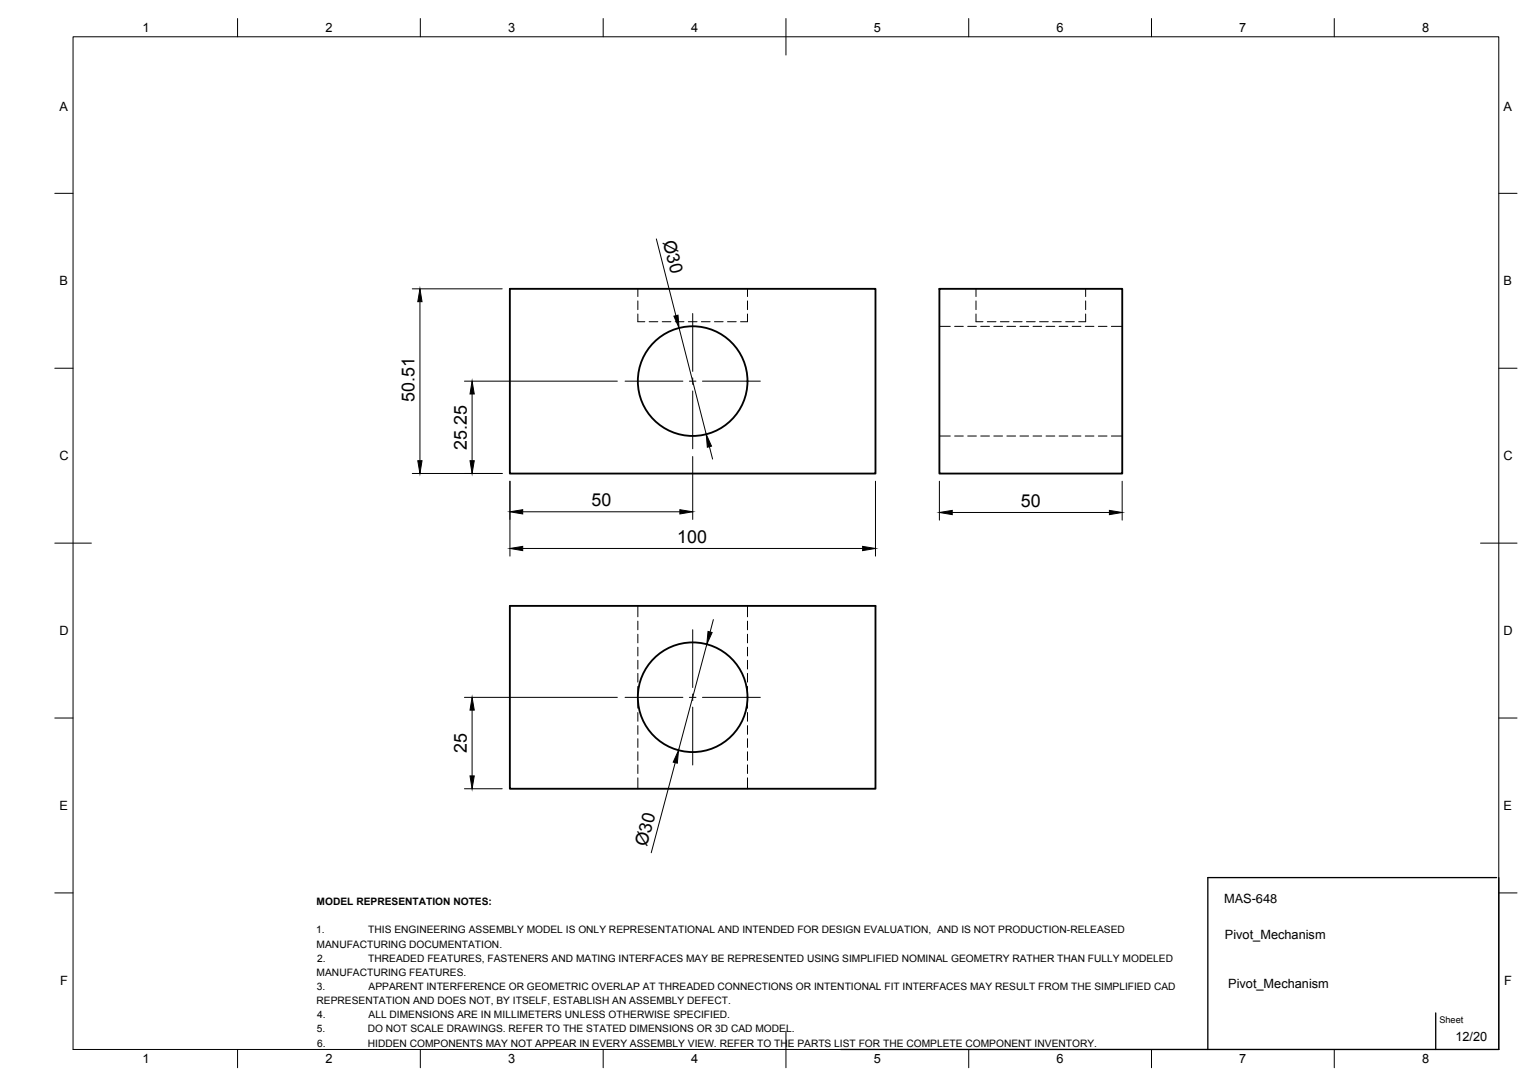
ISO-10303-21;
HEADER;
FILE_DESCRIPTION((''),'2;1');
FILE_NAME('Pivot_Mechanism.step','2026-10-09T12:47:58-07:00',(''),(''),'','','');
FILE_SCHEMA (('AUTOMOTIVE_DESIGN { 1 0 10303 214 3 1 1 }'));
ENDSEC;
DATA;
#10=MECHANICAL_DESIGN_GEOMETRIC_PRESENTATION_REPRESENTATION('',(#315),#3475);
#148=FACE_BOUND('',#494,.T.) ;
#149=FACE_BOUND('',#497,.T.) ;
#150=FACE_BOUND('',#499,.T.) ;
#178=CIRCLE('',#2031,15.) ;
#179=CIRCLE('',#2032,15.) ;
#180=CIRCLE('',#2034,15.) ;
#181=CIRCLE('',#2035,15.) ;
#263=CYLINDRICAL_SURFACE('',#2030,15.) ;
#264=CYLINDRICAL_SURFACE('',#2033,15.) ;
#291=SHAPE_REPRESENTATION_RELATIONSHIP('SRR','None',#3546,#303) ;
#303=ADVANCED_BREP_SHAPE_REPRESENTATION('',(#327),#3466) ;
#315=STYLED_ITEM('',(#3628),#327) ;
#327=MANIFOLD_SOLID_BREP('Body1',#1829) ;
#370=FACE_OUTER_BOUND('',#491,.T.) ;
#371=FACE_OUTER_BOUND('',#492,.T.) ;
#372=FACE_OUTER_BOUND('',#493,.T.) ;
#373=FACE_OUTER_BOUND('',#495,.T.) ;
#374=FACE_OUTER_BOUND('',#496,.T.) ;
#375=FACE_OUTER_BOUND('',#498,.T.) ;
#376=FACE_OUTER_BOUND('',#500,.T.) ;
#377=FACE_OUTER_BOUND('',#501,.T.) ;
#378=FACE_OUTER_BOUND('',#502,.T.) ;
#491=EDGE_LOOP('',(#1352,#1353,#1354,#1355)) ;
#492=EDGE_LOOP('',(#1356,#1357,#1358,#1359)) ;
#493=EDGE_LOOP('',(#1360,#1361,#1362,#1363)) ;
#494=EDGE_LOOP('',(#1364)) ;
#495=EDGE_LOOP('',(#1365,#1366,#1367,#1368)) ;
#496=EDGE_LOOP('',(#1369,#1370,#1371,#1372)) ;
#497=EDGE_LOOP('',(#1373)) ;
#498=EDGE_LOOP('',(#1374,#1375,#1376,#1377)) ;
#499=EDGE_LOOP('',(#1378)) ;
#500=EDGE_LOOP('',(#1379,#1380,#1381,#1382)) ;
#501=EDGE_LOOP('',(#1383,#1384,#1385,#1386)) ;
#502=EDGE_LOOP('',(#1387)) ;
#650=LINE('',#3076,#769) ;
#651=LINE('',#3082,#770) ;
#652=LINE('',#3087,#771) ;
#653=LINE('',#3089,#772) ;
#654=LINE('',#3091,#773) ;
#655=LINE('',#3092,#774) ;
#656=LINE('',#3095,#775) ;
#657=LINE('',#3097,#776) ;
#658=LINE('',#3098,#777) ;
#659=LINE('',#3101,#778) ;
#660=LINE('',#3103,#779) ;
#661=LINE('',#3104,#780) ;
#662=LINE('',#3106,#781) ;
#663=LINE('',#3107,#782) ;
#769=VECTOR('',#2403,15.) ;
#770=VECTOR('',#2410,15.) ;
#771=VECTOR('',#2415,1000.) ;
#772=VECTOR('',#2416,1000.) ;
#773=VECTOR('',#2417,1000.) ;
#774=VECTOR('',#2418,1000.) ;
#775=VECTOR('',#2421,1000.) ;
#776=VECTOR('',#2422,1000.) ;
#777=VECTOR('',#2423,1000.) ;
#778=VECTOR('',#2426,1000.) ;
#779=VECTOR('',#2427,1000.) ;
#780=VECTOR('',#2428,1000.) ;
#781=VECTOR('',#2431,1000.) ;
#782=VECTOR('',#2432,1000.) ;
#877=VERTEX_POINT('',#3073) ;
#878=VERTEX_POINT('',#3075) ;
#879=VERTEX_POINT('',#3079) ;
#880=VERTEX_POINT('',#3081) ;
#881=VERTEX_POINT('',#3085) ;
#882=VERTEX_POINT('',#3086) ;
#883=VERTEX_POINT('',#3088) ;
#884=VERTEX_POINT('',#3090) ;
#885=VERTEX_POINT('',#3094) ;
#886=VERTEX_POINT('',#3096) ;
#887=VERTEX_POINT('',#3100) ;
#888=VERTEX_POINT('',#3102) ;
#1048=EDGE_CURVE('',#877,#877,#178,.T.) ;
#1049=EDGE_CURVE('',#877,#878,#650,.T.) ;
#1050=EDGE_CURVE('',#878,#878,#179,.T.) ;
#1051=EDGE_CURVE('',#879,#879,#180,.T.) ;
#1052=EDGE_CURVE('',#879,#880,#651,.T.) ;
#1053=EDGE_CURVE('',#880,#880,#181,.T.) ;
#1054=EDGE_CURVE('',#881,#882,#652,.T.) ;
#1055=EDGE_CURVE('',#883,#882,#653,.T.) ;
#1056=EDGE_CURVE('',#884,#883,#654,.T.) ;
#1057=EDGE_CURVE('',#884,#881,#655,.T.) ;
#1058=EDGE_CURVE('',#882,#885,#656,.T.) ;
#1059=EDGE_CURVE('',#886,#885,#657,.T.) ;
#1060=EDGE_CURVE('',#883,#886,#658,.T.) ;
#1061=EDGE_CURVE('',#885,#887,#659,.T.) ;
#1062=EDGE_CURVE('',#888,#887,#660,.T.) ;
#1063=EDGE_CURVE('',#886,#888,#661,.T.) ;
#1064=EDGE_CURVE('',#887,#881,#662,.T.) ;
#1065=EDGE_CURVE('',#888,#884,#663,.T.) ;
#1352=ORIENTED_EDGE('',*,*,#1048,.F.) ;
#1353=ORIENTED_EDGE('',*,*,#1049,.T.) ;
#1354=ORIENTED_EDGE('',*,*,#1050,.T.) ;
#1355=ORIENTED_EDGE('',*,*,#1049,.F.) ;
#1356=ORIENTED_EDGE('',*,*,#1051,.F.) ;
#1357=ORIENTED_EDGE('',*,*,#1052,.T.) ;
#1358=ORIENTED_EDGE('',*,*,#1053,.T.) ;
#1359=ORIENTED_EDGE('',*,*,#1052,.F.) ;
#1360=ORIENTED_EDGE('',*,*,#1054,.T.) ;
#1361=ORIENTED_EDGE('',*,*,#1055,.F.) ;
#1362=ORIENTED_EDGE('',*,*,#1056,.F.) ;
#1363=ORIENTED_EDGE('',*,*,#1057,.T.) ;
#1364=ORIENTED_EDGE('',*,*,#1048,.T.) ;
#1365=ORIENTED_EDGE('',*,*,#1058,.T.) ;
#1366=ORIENTED_EDGE('',*,*,#1059,.F.) ;
#1367=ORIENTED_EDGE('',*,*,#1060,.F.) ;
#1368=ORIENTED_EDGE('',*,*,#1055,.T.) ;
#1369=ORIENTED_EDGE('',*,*,#1061,.T.) ;
#1370=ORIENTED_EDGE('',*,*,#1062,.F.) ;
#1371=ORIENTED_EDGE('',*,*,#1063,.F.) ;
#1372=ORIENTED_EDGE('',*,*,#1059,.T.) ;
#1373=ORIENTED_EDGE('',*,*,#1050,.F.) ;
#1374=ORIENTED_EDGE('',*,*,#1064,.T.) ;
#1375=ORIENTED_EDGE('',*,*,#1057,.F.) ;
#1376=ORIENTED_EDGE('',*,*,#1065,.F.) ;
#1377=ORIENTED_EDGE('',*,*,#1062,.T.) ;
#1378=ORIENTED_EDGE('',*,*,#1053,.F.) ;
#1379=ORIENTED_EDGE('',*,*,#1056,.T.) ;
#1380=ORIENTED_EDGE('',*,*,#1060,.T.) ;
#1381=ORIENTED_EDGE('',*,*,#1063,.T.) ;
#1382=ORIENTED_EDGE('',*,*,#1065,.T.) ;
#1383=ORIENTED_EDGE('',*,*,#1054,.F.) ;
#1384=ORIENTED_EDGE('',*,*,#1064,.F.) ;
#1385=ORIENTED_EDGE('',*,*,#1061,.F.) ;
#1386=ORIENTED_EDGE('',*,*,#1058,.F.) ;
#1387=ORIENTED_EDGE('',*,*,#1051,.T.) ;
#1672=PLANE('',#2036) ;
#1673=PLANE('',#2037) ;
#1674=PLANE('',#2038) ;
#1675=PLANE('',#2039) ;
#1676=PLANE('',#2040) ;
#1677=PLANE('',#2041) ;
#1678=PLANE('',#2042) ;
#1746=ADVANCED_FACE('',(#370),#263,.F.) ;
#1747=ADVANCED_FACE('',(#371),#264,.F.) ;
#1748=ADVANCED_FACE('',(#372,#148),#1672,.F.) ;
#1749=ADVANCED_FACE('',(#373),#1673,.F.) ;
#1750=ADVANCED_FACE('',(#374,#149),#1674,.F.) ;
#1751=ADVANCED_FACE('',(#375,#150),#1675,.F.) ;
#1752=ADVANCED_FACE('',(#376),#1676,.T.) ;
#1753=ADVANCED_FACE('',(#377),#1677,.F.) ;
#1754=ADVANCED_FACE('',(#378),#1678,.T.) ;
#1829=CLOSED_SHELL('',(#1746,#1747,#1748,#1749,#1750,#1751,#1752,#1753,
#1754)) ;
#2029=AXIS2_PLACEMENT_3D('',#3071,#2397,#2398) ;
#2030=AXIS2_PLACEMENT_3D('',#3072,#2399,#2400) ;
#2031=AXIS2_PLACEMENT_3D('',#3074,#2401,#2402) ;
#2032=AXIS2_PLACEMENT_3D('',#3077,#2404,#2405) ;
#2033=AXIS2_PLACEMENT_3D('',#3078,#2406,#2407) ;
#2034=AXIS2_PLACEMENT_3D('',#3080,#2408,#2409) ;
#2035=AXIS2_PLACEMENT_3D('',#3083,#2411,#2412) ;
#2036=AXIS2_PLACEMENT_3D('',#3084,#2413,#2414) ;
#2037=AXIS2_PLACEMENT_3D('',#3093,#2419,#2420) ;
#2038=AXIS2_PLACEMENT_3D('',#3099,#2424,#2425) ;
#2039=AXIS2_PLACEMENT_3D('',#3105,#2429,#2430) ;
#2040=AXIS2_PLACEMENT_3D('',#3108,#2433,#2434) ;
#2041=AXIS2_PLACEMENT_3D('',#3109,#2435,#2436) ;
#2042=AXIS2_PLACEMENT_3D('',#3110,#2437,#2438) ;
#2397=DIRECTION('axis',(0.,0.,1.)) ;
#2398=DIRECTION('refdir',(1.,0.,0.)) ;
#2399=DIRECTION('center_axis',(1.,0.,0.)) ;
#2400=DIRECTION('ref_axis',(0.,0.,-1.)) ;
#2401=DIRECTION('center_axis',(1.,0.,0.)) ;
#2402=DIRECTION('ref_axis',(0.,0.,-1.)) ;
#2403=DIRECTION('',(1.,0.,0.)) ;
#2404=DIRECTION('center_axis',(1.,0.,0.)) ;
#2405=DIRECTION('ref_axis',(0.,0.,-1.)) ;
#2406=DIRECTION('center_axis',(0.,1.,0.)) ;
#2407=DIRECTION('ref_axis',(0.,0.,1.)) ;
#2408=DIRECTION('center_axis',(0.,1.,0.)) ;
#2409=DIRECTION('ref_axis',(0.,0.,1.)) ;
#2410=DIRECTION('',(0.,1.,0.)) ;
#2411=DIRECTION('center_axis',(0.,1.,0.)) ;
#2412=DIRECTION('ref_axis',(0.,0.,1.)) ;
#2413=DIRECTION('center_axis',(1.,0.,0.)) ;
#2414=DIRECTION('ref_axis',(0.,0.,-1.)) ;
#2415=DIRECTION('',(0.,-1.,0.)) ;
#2416=DIRECTION('',(0.,0.,-1.)) ;
#2417=DIRECTION('',(0.,-1.,0.)) ;
#2418=DIRECTION('',(0.,0.,-1.)) ;
#2419=DIRECTION('center_axis',(0.,1.,0.)) ;
#2420=DIRECTION('ref_axis',(0.,0.,1.)) ;
#2421=DIRECTION('',(1.,0.,0.)) ;
#2422=DIRECTION('',(0.,0.,-1.)) ;
#2423=DIRECTION('',(1.,0.,0.)) ;
#2424=DIRECTION('center_axis',(-1.,0.,0.)) ;
#2425=DIRECTION('ref_axis',(0.,0.,1.)) ;
#2426=DIRECTION('',(0.,1.,0.)) ;
#2427=DIRECTION('',(0.,0.,-1.)) ;
#2428=DIRECTION('',(0.,1.,0.)) ;
#2429=DIRECTION('center_axis',(0.,-1.,0.)) ;
#2430=DIRECTION('ref_axis',(0.,0.,-1.)) ;
#2431=DIRECTION('',(-1.,0.,0.)) ;
#2432=DIRECTION('',(-1.,0.,0.)) ;
#2433=DIRECTION('center_axis',(0.,0.,1.)) ;
#2434=DIRECTION('ref_axis',(1.,0.,0.)) ;
#2435=DIRECTION('center_axis',(0.,0.,1.)) ;
#2436=DIRECTION('ref_axis',(1.,0.,0.)) ;
#2437=DIRECTION('center_axis',(0.,1.,0.)) ;
#2438=DIRECTION('ref_axis',(0.,0.,1.)) ;
#3071=CARTESIAN_POINT('',(0.,0.,0.)) ;
#3072=CARTESIAN_POINT('Origin',(-25.,0.,0.)) ;
#3073=CARTESIAN_POINT('',(-25.,-1.83697019872103E-15,15.)) ;
#3074=CARTESIAN_POINT('Origin',(-25.,0.,0.)) ;
#3075=CARTESIAN_POINT('',(25.,-1.83697019872103E-15,15.)) ;
#3076=CARTESIAN_POINT('',(-25.,-1.83697019872103E-15,15.)) ;
#3077=CARTESIAN_POINT('Origin',(25.,0.,0.)) ;
#3078=CARTESIAN_POINT('Origin',(0.,16.254058593968,0.)) ;
#3079=CARTESIAN_POINT('',(-1.83697019872103E-15,16.254058593968,-15.)) ;
#3080=CARTESIAN_POINT('Origin',(0.,16.254058593968,0.)) ;
#3081=CARTESIAN_POINT('',(-1.83697019872103E-15,25.254058593968,-15.)) ;
#3082=CARTESIAN_POINT('',(-1.83697019872103E-15,16.254058593968,-15.)) ;
#3083=CARTESIAN_POINT('Origin',(0.,25.254058593968,0.)) ;
#3084=CARTESIAN_POINT('Origin',(-25.,-25.254058593968,50.)) ;
#3085=CARTESIAN_POINT('',(-25.,25.254058593968,-50.)) ;
#3086=CARTESIAN_POINT('',(-25.,-25.254058593968,-50.)) ;
#3087=CARTESIAN_POINT('',(-25.,-25.254058593968,-50.)) ;
#3088=CARTESIAN_POINT('',(-25.,-25.254058593968,50.)) ;
#3089=CARTESIAN_POINT('',(-25.,-25.254058593968,50.)) ;
#3090=CARTESIAN_POINT('',(-25.,25.254058593968,50.)) ;
#3091=CARTESIAN_POINT('',(-25.,-25.254058593968,50.)) ;
#3092=CARTESIAN_POINT('',(-25.,25.254058593968,50.)) ;
#3093=CARTESIAN_POINT('Origin',(25.,-25.254058593968,50.)) ;
#3094=CARTESIAN_POINT('',(25.,-25.254058593968,-50.)) ;
#3095=CARTESIAN_POINT('',(25.,-25.254058593968,-50.)) ;
#3096=CARTESIAN_POINT('',(25.,-25.254058593968,50.)) ;
#3097=CARTESIAN_POINT('',(25.,-25.254058593968,50.)) ;
#3098=CARTESIAN_POINT('',(25.,-25.254058593968,50.)) ;
#3099=CARTESIAN_POINT('Origin',(25.,-25.254058593968,50.)) ;
#3100=CARTESIAN_POINT('',(25.,25.254058593968,-50.)) ;
#3101=CARTESIAN_POINT('',(25.,-25.254058593968,-50.)) ;
#3102=CARTESIAN_POINT('',(25.,25.254058593968,50.)) ;
#3103=CARTESIAN_POINT('',(25.,25.254058593968,50.)) ;
#3104=CARTESIAN_POINT('',(25.,-25.254058593968,50.)) ;
#3105=CARTESIAN_POINT('Origin',(25.,25.254058593968,50.)) ;
#3106=CARTESIAN_POINT('',(25.,25.254058593968,-50.)) ;
#3107=CARTESIAN_POINT('',(25.,25.254058593968,50.)) ;
#3108=CARTESIAN_POINT('Origin',(0.,0.,50.)) ;
#3109=CARTESIAN_POINT('Origin',(0.,0.,-50.)) ;
#3110=CARTESIAN_POINT('Origin',(0.,16.254058593968,0.)) ;
#3448=UNCERTAINTY_MEASURE_WITH_UNIT(LENGTH_MEASURE(0.01),#3476,
'DISTANCE_ACCURACY_VALUE',
'Maximum model space distance between geometric entities at asserted c
onnectivities') ;
#3457=UNCERTAINTY_MEASURE_WITH_UNIT(LENGTH_MEASURE(0.01),#3476,
'DISTANCE_ACCURACY_VALUE',
'Maximum model space distance between geometric entities at asserted c
onnectivities') ;
#3466=(
GEOMETRIC_REPRESENTATION_CONTEXT(3)
GLOBAL_UNCERTAINTY_ASSIGNED_CONTEXT((#3448))
GLOBAL_UNIT_ASSIGNED_CONTEXT((#3476,#3478,#3479))
REPRESENTATION_CONTEXT('','3D')
) ;
#3475=(
GEOMETRIC_REPRESENTATION_CONTEXT(3)
GLOBAL_UNCERTAINTY_ASSIGNED_CONTEXT((#3457))
GLOBAL_UNIT_ASSIGNED_CONTEXT((#3476,#3478,#3479))
REPRESENTATION_CONTEXT('','3D')
) ;
#3476=(
LENGTH_UNIT()
NAMED_UNIT(*)
SI_UNIT(.MILLI.,.METRE.)
) ;
#3478=(
NAMED_UNIT(*)
PLANE_ANGLE_UNIT()
SI_UNIT($,.RADIAN.)
) ;
#3479=(
NAMED_UNIT(*)
SI_UNIT($,.STERADIAN.)
SOLID_ANGLE_UNIT()
) ;
#3488=SHAPE_DEFINITION_REPRESENTATION(#3509,#3546) ;
#3509=PRODUCT_DEFINITION_SHAPE('',$,#3564) ;
#3546=SHAPE_REPRESENTATION('',(#2029),#3466) ;
#3555=PRODUCT_DEFINITION_CONTEXT('part definition',#3608,'design') ;
#3564=PRODUCT_DEFINITION('Pivot_Mechanism','Pivot_Mechanism',#3581,#3555) ;
#3581=PRODUCT_DEFINITION_FORMATION('',$,#3618) ;
#3608=APPLICATION_CONTEXT(
'Core Data for Automotive Mechanical Design Process') ;
#3609=PRODUCT_CONTEXT('part definition',#3608,'mechanical') ;
#3618=PRODUCT('Pivot_Mechanism',
'Pivot_Mechanism',$,(#3609)) ;
#3628=PRESENTATION_STYLE_ASSIGNMENT((#3630)) ;
#3630=SURFACE_STYLE_USAGE(.BOTH.,#3632) ;
#3632=SURFACE_SIDE_STYLE('',(#3634)) ;
#3634=SURFACE_STYLE_FILL_AREA(#3636) ;
#3636=FILL_AREA_STYLE('Opaque(202,209,238)',(#3638)) ;
#3638=FILL_AREA_STYLE_COLOUR('Opaque(202,209,238)',#3640) ;
#3640=COLOUR_RGB('Opaque(202,209,238)', 0.09019608, 0.27058824, 0.51372549) ;
ENDSEC;
END-ISO-10303-21;
